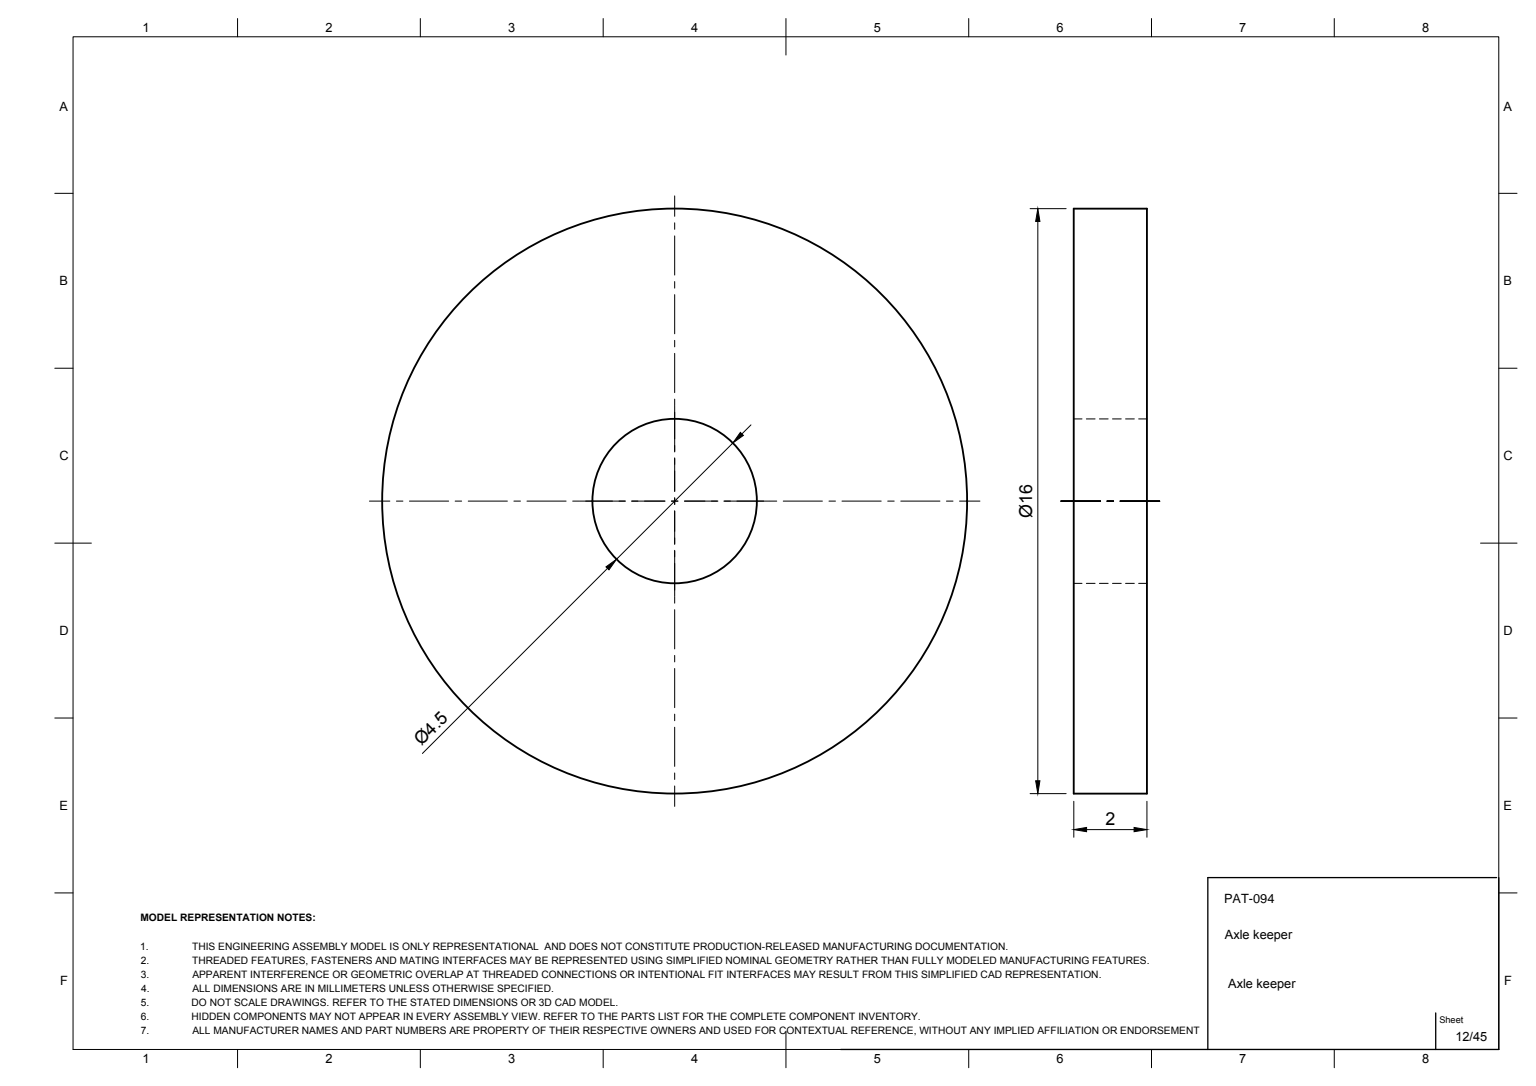
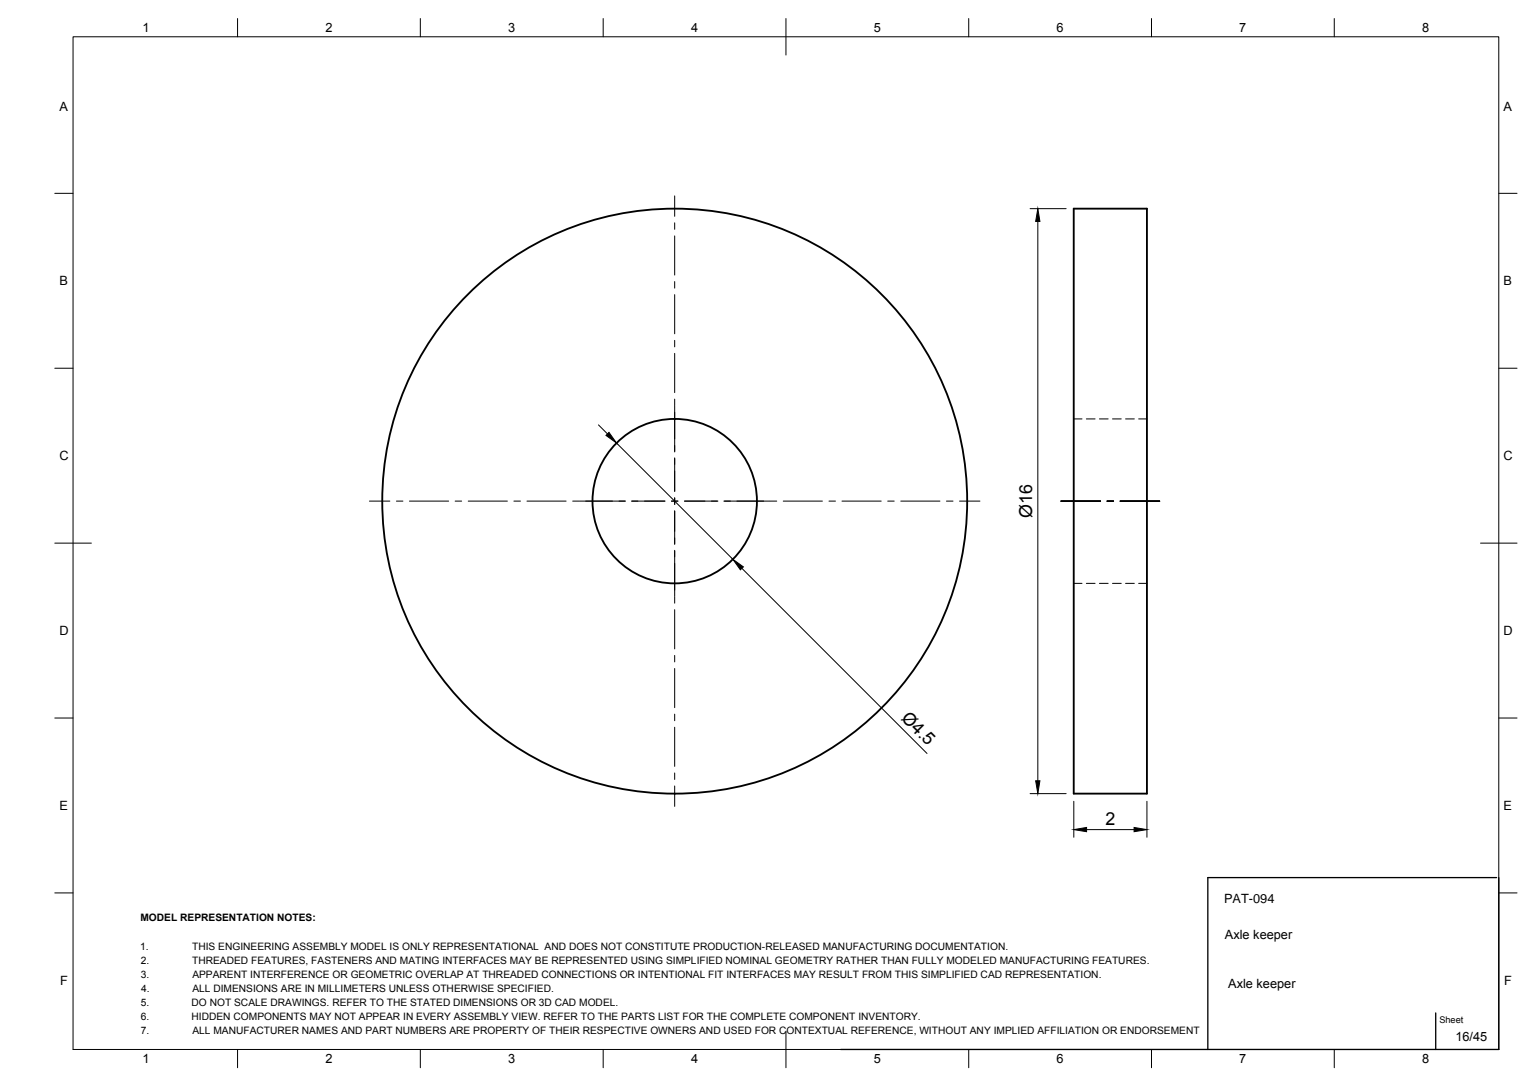
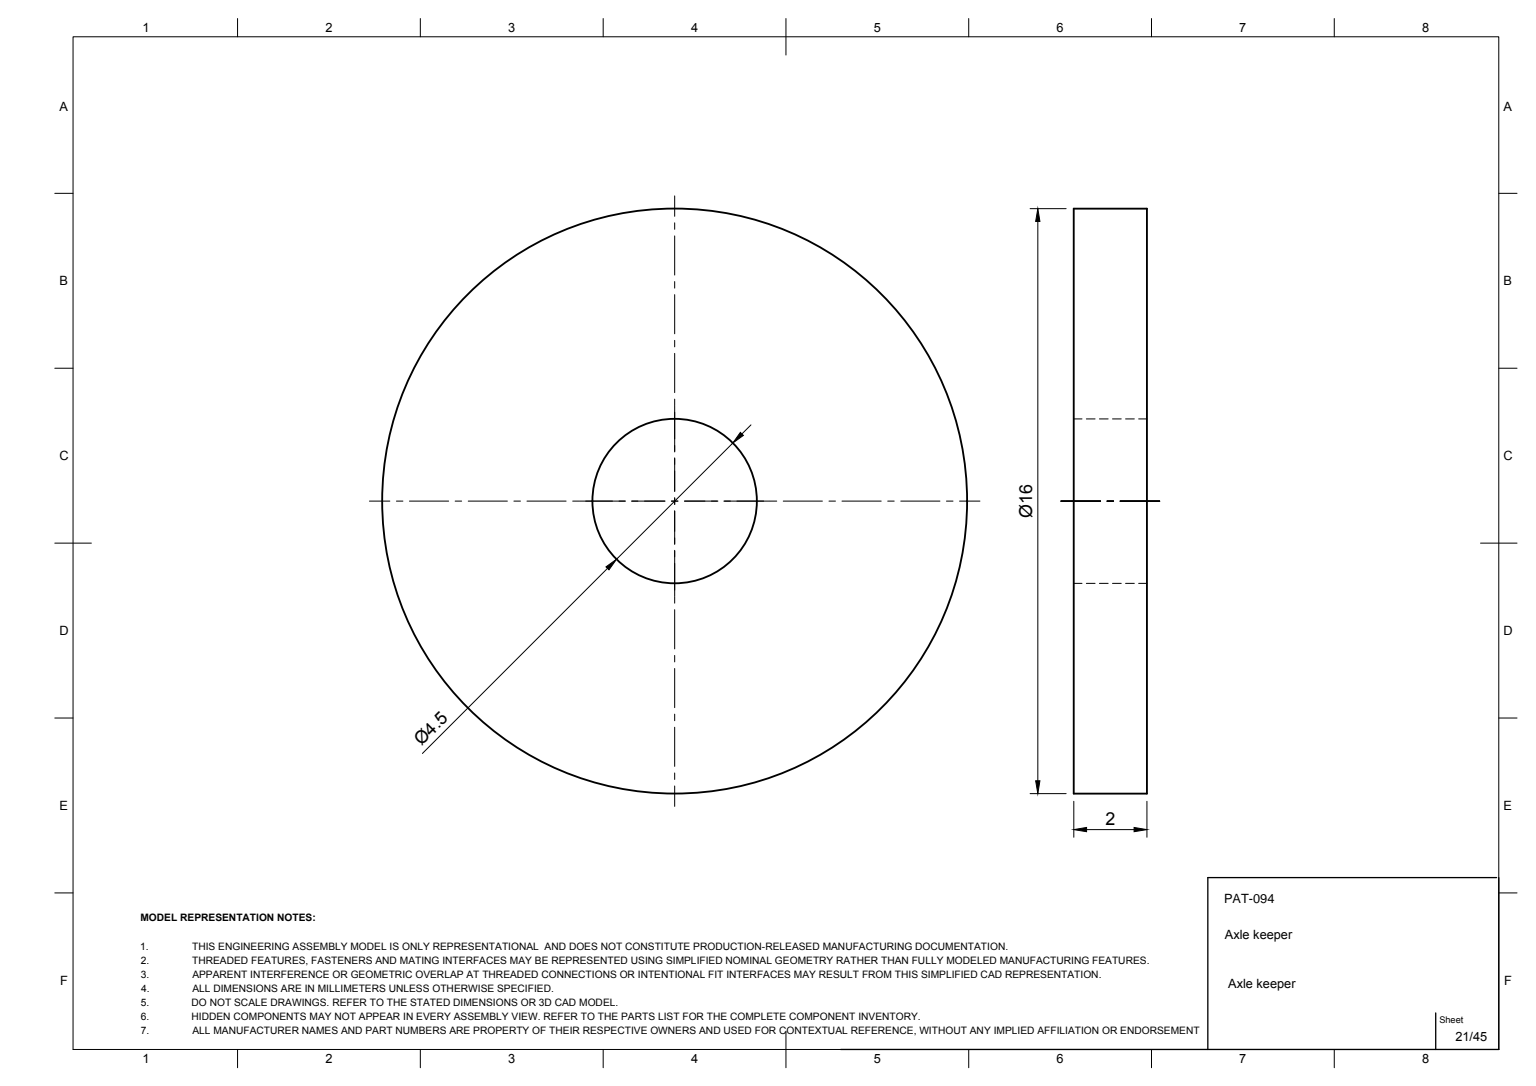
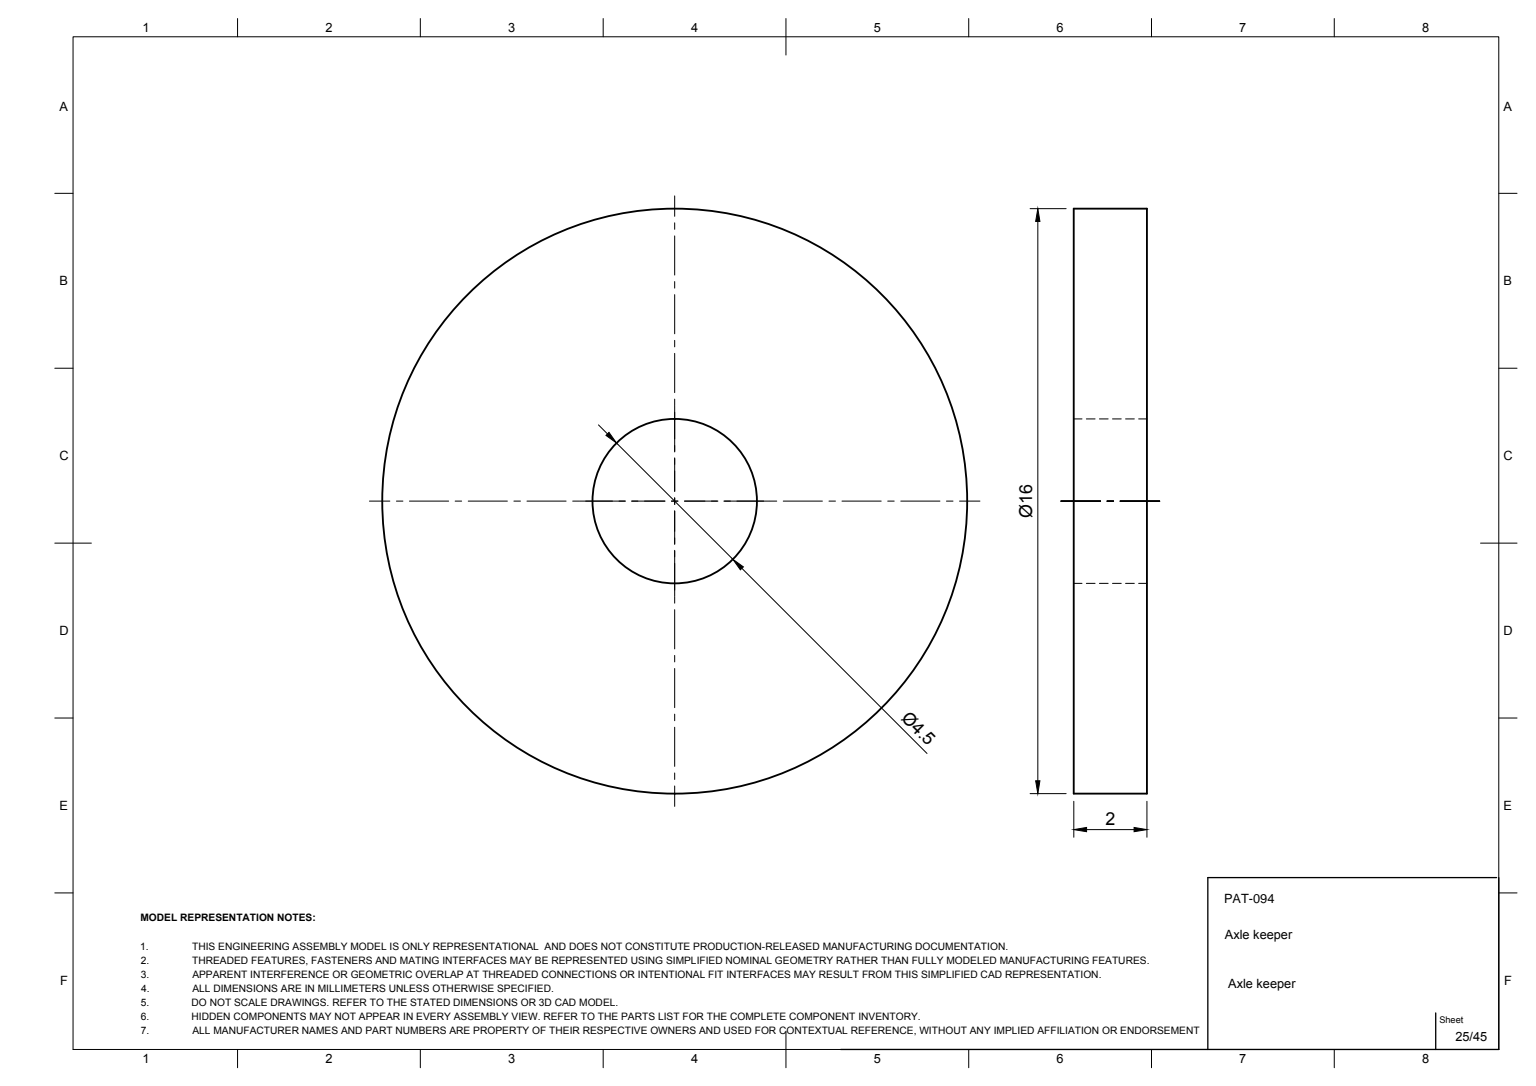
ISO-10303-21;
HEADER;
/* Generated by software containing ST-Developer
 * from STEP Tools, Inc. (www.steptools.com) 
 */

FILE_DESCRIPTION(
/* description */ ('Shaft runout checking stand'),
/* implementation_level */ '2;1');

FILE_NAME(
/* name */ 'Axle keeper.step',
/* time_stamp */ '2026-11-02T21:12:33-08:00',
/* author */ (''),
/* organization */ (''),
/* preprocessor_version */ 'ST-DEVELOPER v20.2',
/* originating_system */ 'Autodesk Translation Framework v15.17.0.0',
/* authorisation */ '');

FILE_SCHEMA (('AUTOMOTIVE_DESIGN { 1 0 10303 214 3 1 1 }'));
ENDSEC;

DATA;
#10=MECHANICAL_DESIGN_GEOMETRIC_PRESENTATION_REPRESENTATION('',(#473),#11748);
#387=SHAPE_REPRESENTATION_RELATIONSHIP('SRR','None',#11936,#430);
#430=ADVANCED_BREP_SHAPE_REPRESENTATION('',(#524),#11712);
#473=STYLED_ITEM('',(#12169),#524);
#524=MANIFOLD_SOLID_BREP('Body1',#6216);
#605=FACE_BOUND('',#1577,.T.);
#606=FACE_BOUND('',#1579,.T.);
#732=CIRCLE('',#6934,0.225);
#733=CIRCLE('',#6935,0.225);
#734=CIRCLE('',#6937,0.8);
#735=CIRCLE('',#6938,0.8);
#966=CYLINDRICAL_SURFACE('',#6933,0.225);
#967=CYLINDRICAL_SURFACE('',#6936,0.8);
#1163=FACE_OUTER_BOUND('',#1574,.T.);
#1164=FACE_OUTER_BOUND('',#1575,.T.);
#1165=FACE_OUTER_BOUND('',#1576,.T.);
#1166=FACE_OUTER_BOUND('',#1578,.T.);
#1574=EDGE_LOOP('',(#4710,#4711,#4712,#4713));
#1575=EDGE_LOOP('',(#4714,#4715,#4716,#4717));
#1576=EDGE_LOOP('',(#4718));
#1577=EDGE_LOOP('',(#4719));
#1578=EDGE_LOOP('',(#4720));
#1579=EDGE_LOOP('',(#4721));
#2135=LINE('',#10135,#2602);
#2136=LINE('',#10141,#2603);
#2602=VECTOR('',#8144,0.225);
#2603=VECTOR('',#8151,0.8);
#3026=VERTEX_POINT('',#10132);
#3027=VERTEX_POINT('',#10134);
#3028=VERTEX_POINT('',#10138);
#3029=VERTEX_POINT('',#10140);
#3641=EDGE_CURVE('',#3026,#3026,#732,.T.);
#3642=EDGE_CURVE('',#3026,#3027,#2135,.T.);
#3643=EDGE_CURVE('',#3027,#3027,#733,.T.);
#3644=EDGE_CURVE('',#3028,#3028,#734,.T.);
#3645=EDGE_CURVE('',#3028,#3029,#2136,.T.);
#3646=EDGE_CURVE('',#3029,#3029,#735,.T.);
#4710=ORIENTED_EDGE('',*,*,#3641,.F.);
#4711=ORIENTED_EDGE('',*,*,#3642,.T.);
#4712=ORIENTED_EDGE('',*,*,#3643,.T.);
#4713=ORIENTED_EDGE('',*,*,#3642,.F.);
#4714=ORIENTED_EDGE('',*,*,#3644,.F.);
#4715=ORIENTED_EDGE('',*,*,#3645,.T.);
#4716=ORIENTED_EDGE('',*,*,#3646,.T.);
#4717=ORIENTED_EDGE('',*,*,#3645,.F.);
#4718=ORIENTED_EDGE('',*,*,#3644,.T.);
#4719=ORIENTED_EDGE('',*,*,#3641,.T.);
#4720=ORIENTED_EDGE('',*,*,#3646,.F.);
#4721=ORIENTED_EDGE('',*,*,#3643,.F.);
#5700=PLANE('',#6939);
#5701=PLANE('',#6940);
#5963=ADVANCED_FACE('',(#1163),#966,.F.);
#5964=ADVANCED_FACE('',(#1164),#967,.T.);
#5965=ADVANCED_FACE('',(#1165,#605),#5700,.T.);
#5966=ADVANCED_FACE('',(#1166,#606),#5701,.F.);
#6216=CLOSED_SHELL('',(#5963,#5964,#5965,#5966));
#6932=AXIS2_PLACEMENT_3D('',#10130,#8138,#8139);
#6933=AXIS2_PLACEMENT_3D('',#10131,#8140,#8141);
#6934=AXIS2_PLACEMENT_3D('',#10133,#8142,#8143);
#6935=AXIS2_PLACEMENT_3D('',#10136,#8145,#8146);
#6936=AXIS2_PLACEMENT_3D('',#10137,#8147,#8148);
#6937=AXIS2_PLACEMENT_3D('',#10139,#8149,#8150);
#6938=AXIS2_PLACEMENT_3D('',#10142,#8152,#8153);
#6939=AXIS2_PLACEMENT_3D('',#10143,#8154,#8155);
#6940=AXIS2_PLACEMENT_3D('',#10144,#8156,#8157);
#8138=DIRECTION('axis',(0.,0.,1.));
#8139=DIRECTION('refdir',(1.,0.,0.));
#8140=DIRECTION('center_axis',(0.,1.,0.));
#8141=DIRECTION('ref_axis',(1.,0.,0.));
#8142=DIRECTION('center_axis',(0.,-1.,0.));
#8143=DIRECTION('ref_axis',(1.,0.,0.));
#8144=DIRECTION('',(0.,-1.,0.));
#8145=DIRECTION('center_axis',(0.,-1.,0.));
#8146=DIRECTION('ref_axis',(1.,0.,0.));
#8147=DIRECTION('center_axis',(0.,1.,0.));
#8148=DIRECTION('ref_axis',(1.,0.,0.));
#8149=DIRECTION('center_axis',(0.,1.,0.));
#8150=DIRECTION('ref_axis',(1.,0.,0.));
#8151=DIRECTION('',(0.,-1.,0.));
#8152=DIRECTION('center_axis',(0.,1.,0.));
#8153=DIRECTION('ref_axis',(1.,0.,0.));
#8154=DIRECTION('center_axis',(0.,1.,0.));
#8155=DIRECTION('ref_axis',(1.,0.,0.));
#8156=DIRECTION('center_axis',(0.,1.,0.));
#8157=DIRECTION('ref_axis',(1.,0.,0.));
#10130=CARTESIAN_POINT('',(0.,0.,0.));
#10131=CARTESIAN_POINT('Origin',(-2.,-9.2,5.));
#10132=CARTESIAN_POINT('',(-2.225,-9.,5.));
#10133=CARTESIAN_POINT('Origin',(-2.,-9.,5.));
#10134=CARTESIAN_POINT('',(-2.225,-9.2,5.));
#10135=CARTESIAN_POINT('',(-2.225,-9.2,5.));
#10136=CARTESIAN_POINT('Origin',(-2.,-9.2,5.));
#10137=CARTESIAN_POINT('Origin',(-2.,-9.2,5.));
#10138=CARTESIAN_POINT('',(-2.8,-9.,5.));
#10139=CARTESIAN_POINT('Origin',(-2.,-9.,5.));
#10140=CARTESIAN_POINT('',(-2.8,-9.2,5.));
#10141=CARTESIAN_POINT('',(-2.8,-9.2,5.));
#10142=CARTESIAN_POINT('Origin',(-2.,-9.2,5.));
#10143=CARTESIAN_POINT('Origin',(-2.,-9.,5.));
#10144=CARTESIAN_POINT('Origin',(-2.,-9.2,5.));
#11663=UNCERTAINTY_MEASURE_WITH_UNIT(LENGTH_MEASURE(0.001),#11749,
'DISTANCE_ACCURACY_VALUE',
'Maximum model space distance between geometric entities at asserted c
onnectivities');
#11699=UNCERTAINTY_MEASURE_WITH_UNIT(LENGTH_MEASURE(0.001),#11749,
'DISTANCE_ACCURACY_VALUE',
'Maximum model space distance between geometric entities at asserted c
onnectivities');
#11712=(
GEOMETRIC_REPRESENTATION_CONTEXT(3)
GLOBAL_UNCERTAINTY_ASSIGNED_CONTEXT((#11663))
GLOBAL_UNIT_ASSIGNED_CONTEXT((#11749,#11751,#11752))
REPRESENTATION_CONTEXT('','3D')
);
#11748=(
GEOMETRIC_REPRESENTATION_CONTEXT(3)
GLOBAL_UNCERTAINTY_ASSIGNED_CONTEXT((#11699))
GLOBAL_UNIT_ASSIGNED_CONTEXT((#11749,#11751,#11752))
REPRESENTATION_CONTEXT('','3D')
);
#11749=(
LENGTH_UNIT()
NAMED_UNIT(*)
SI_UNIT(.CENTI.,.METRE.)
);
#11751=(
NAMED_UNIT(*)
PLANE_ANGLE_UNIT()
SI_UNIT($,.RADIAN.)
);
#11752=(
NAMED_UNIT(*)
SI_UNIT($,.STERADIAN.)
SOLID_ANGLE_UNIT()
);
#11765=SHAPE_DEFINITION_REPRESENTATION(#11813,#11936);
#11813=PRODUCT_DEFINITION_SHAPE('',$,#11985);
#11936=SHAPE_REPRESENTATION('',(#6932),#11712);
#11972=PRODUCT_DEFINITION_CONTEXT('part definition',#12118,'design');
#11985=PRODUCT_DEFINITION('Axle keeper','Axle keeper',#12033,#11972);
#12033=PRODUCT_DEFINITION_FORMATION('',$,#12132);
#12118=APPLICATION_CONTEXT(
'Core Data for Automotive Mechanical Design Process');
#12119=PRODUCT_CONTEXT('part definition',#12118,'mechanical');
#12132=PRODUCT('Axle keeper','Axle keeper','Axle keeper',(#12119));
#12169=PRESENTATION_STYLE_ASSIGNMENT((#12174));
#12174=SURFACE_STYLE_USAGE(.BOTH.,#12179);
#12179=SURFACE_SIDE_STYLE('',(#12184));
#12184=SURFACE_STYLE_FILL_AREA(#12189);
#12189=FILL_AREA_STYLE('CAD Library Painted - Engineering blue',(#12194));
#12194=FILL_AREA_STYLE_COLOUR('CAD Library Painted - Engineering blue',
#12199);
#12199=COLOUR_RGB('CAD Library Painted - Engineering blue',0.12156862745098,
0.356862745098039,0.6);
ENDSEC;
END-ISO-10303-21;
